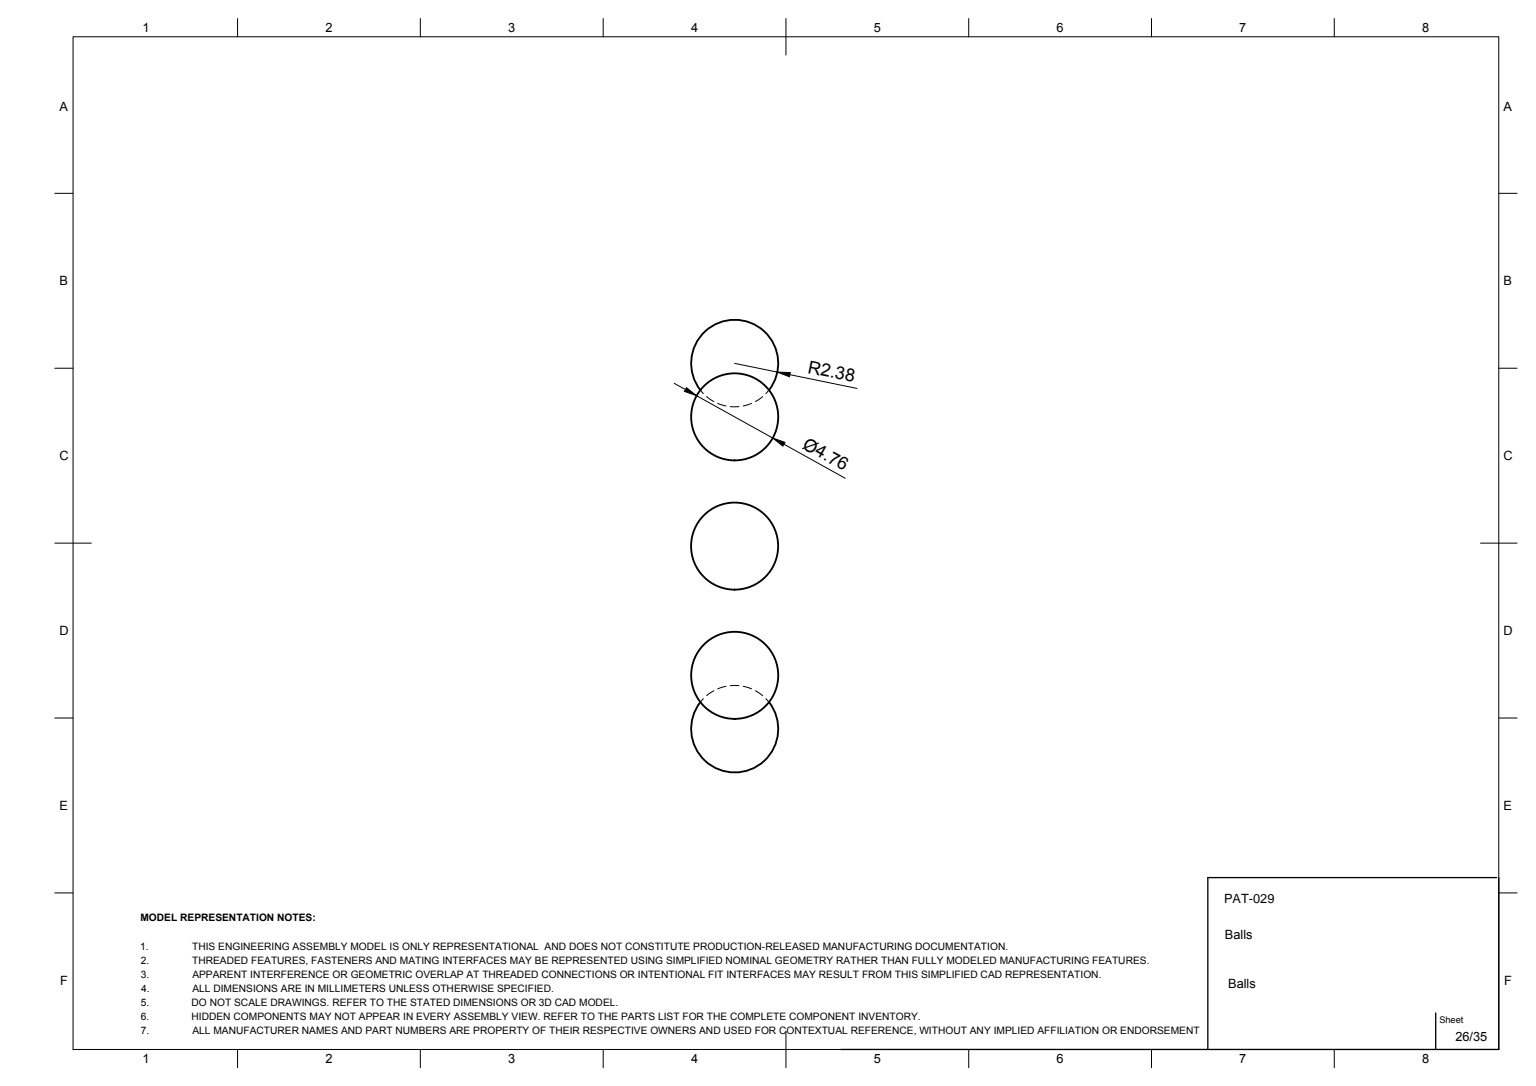
ISO-10303-21;
HEADER;
/* Generated by software containing ST-Developer
 * from STEP Tools, Inc. (www.steptools.com) 
 */

FILE_DESCRIPTION(
/* description */ ('Door-style hinge test fixture with detent'),
/* implementation_level */ '2;1');

FILE_NAME(
/* name */ 'Balls.step',
/* time_stamp */ '2026-10-28T03:24:57-07:00',
/* author */ (''),
/* organization */ (''),
/* preprocessor_version */ 'ST-DEVELOPER v20.2',
/* originating_system */ 'Autodesk Translation Framework v15.17.0.0',
/* authorisation */ '');

FILE_SCHEMA (('AUTOMOTIVE_DESIGN { 1 0 10303 214 3 1 1 }'));
ENDSEC;

DATA;
#10=MECHANICAL_DESIGN_GEOMETRIC_PRESENTATION_REPRESENTATION('',(#344,#345,#346,#347,#348,#349,#350,#351),#9813);
#243=SPHERICAL_SURFACE('',#5484,0.23815);
#244=SPHERICAL_SURFACE('',#5486,0.23815);
#245=SPHERICAL_SURFACE('',#5488,0.23815);
#246=SPHERICAL_SURFACE('',#5490,0.23815);
#247=SPHERICAL_SURFACE('',#5492,0.23815);
#248=SPHERICAL_SURFACE('',#5494,0.23815);
#249=SPHERICAL_SURFACE('',#5496,0.23815);
#250=SPHERICAL_SURFACE('',#5498,0.23815);
#281=SHAPE_REPRESENTATION_RELATIONSHIP('SRR','None',#9959,#312);
#312=ADVANCED_BREP_SHAPE_REPRESENTATION('',(#383,#384,#385,#386,#387,#388,
#389,#390),#9802);
#344=STYLED_ITEM('',(#10183),#383);
#345=STYLED_ITEM('',(#10183),#384);
#346=STYLED_ITEM('',(#10183),#385);
#347=STYLED_ITEM('',(#10183),#386);
#348=STYLED_ITEM('',(#10183),#387);
#349=STYLED_ITEM('',(#10183),#388);
#350=STYLED_ITEM('',(#10183),#389);
#351=STYLED_ITEM('',(#10183),#390);
#383=MANIFOLD_SOLID_BREP('Body1',#4776);
#384=MANIFOLD_SOLID_BREP('Body2',#4777);
#385=MANIFOLD_SOLID_BREP('Body3',#4778);
#386=MANIFOLD_SOLID_BREP('Body4',#4779);
#387=MANIFOLD_SOLID_BREP('Body5',#4780);
#388=MANIFOLD_SOLID_BREP('Body6',#4781);
#389=MANIFOLD_SOLID_BREP('Body7',#4782);
#390=MANIFOLD_SOLID_BREP('Body8',#4783);
#841=FACE_OUTER_BOUND('',#1199,.T.);
#842=FACE_OUTER_BOUND('',#1200,.T.);
#843=FACE_OUTER_BOUND('',#1201,.T.);
#844=FACE_OUTER_BOUND('',#1202,.T.);
#845=FACE_OUTER_BOUND('',#1203,.T.);
#846=FACE_OUTER_BOUND('',#1204,.T.);
#847=FACE_OUTER_BOUND('',#1205,.T.);
#848=FACE_OUTER_BOUND('',#1206,.T.);
#1199=EDGE_LOOP('',(#3963,#3964));
#1200=EDGE_LOOP('',(#3965,#3966));
#1201=EDGE_LOOP('',(#3967,#3968));
#1202=EDGE_LOOP('',(#3969,#3970));
#1203=EDGE_LOOP('',(#3971,#3972));
#1204=EDGE_LOOP('',(#3973,#3974));
#1205=EDGE_LOOP('',(#3975,#3976));
#1206=EDGE_LOOP('',(#3977,#3978));
#2118=CIRCLE('',#5485,0.23815);
#2119=CIRCLE('',#5487,0.23815);
#2120=CIRCLE('',#5489,0.23815);
#2121=CIRCLE('',#5491,0.23815);
#2122=CIRCLE('',#5493,0.23815);
#2123=CIRCLE('',#5495,0.23815);
#2124=CIRCLE('',#5497,0.23815);
#2125=CIRCLE('',#5499,0.23815);
#2472=VERTEX_POINT('',#8843);
#2473=VERTEX_POINT('',#8844);
#2474=VERTEX_POINT('',#8847);
#2475=VERTEX_POINT('',#8848);
#2476=VERTEX_POINT('',#8851);
#2477=VERTEX_POINT('',#8852);
#2478=VERTEX_POINT('',#8855);
#2479=VERTEX_POINT('',#8856);
#2480=VERTEX_POINT('',#8859);
#2481=VERTEX_POINT('',#8860);
#2482=VERTEX_POINT('',#8863);
#2483=VERTEX_POINT('',#8864);
#2484=VERTEX_POINT('',#8867);
#2485=VERTEX_POINT('',#8868);
#2486=VERTEX_POINT('',#8871);
#2487=VERTEX_POINT('',#8872);
#2998=EDGE_CURVE('',#2472,#2473,#2118,.T.);
#2999=EDGE_CURVE('',#2474,#2475,#2119,.T.);
#3000=EDGE_CURVE('',#2476,#2477,#2120,.T.);
#3001=EDGE_CURVE('',#2478,#2479,#2121,.T.);
#3002=EDGE_CURVE('',#2480,#2481,#2122,.T.);
#3003=EDGE_CURVE('',#2482,#2483,#2123,.T.);
#3004=EDGE_CURVE('',#2484,#2485,#2124,.T.);
#3005=EDGE_CURVE('',#2486,#2487,#2125,.T.);
#3963=ORIENTED_EDGE('',*,*,#2998,.T.);
#3964=ORIENTED_EDGE('',*,*,#2998,.F.);
#3965=ORIENTED_EDGE('',*,*,#2999,.T.);
#3966=ORIENTED_EDGE('',*,*,#2999,.F.);
#3967=ORIENTED_EDGE('',*,*,#3000,.T.);
#3968=ORIENTED_EDGE('',*,*,#3000,.F.);
#3969=ORIENTED_EDGE('',*,*,#3001,.T.);
#3970=ORIENTED_EDGE('',*,*,#3001,.F.);
#3971=ORIENTED_EDGE('',*,*,#3002,.T.);
#3972=ORIENTED_EDGE('',*,*,#3002,.F.);
#3973=ORIENTED_EDGE('',*,*,#3003,.T.);
#3974=ORIENTED_EDGE('',*,*,#3003,.F.);
#3975=ORIENTED_EDGE('',*,*,#3004,.T.);
#3976=ORIENTED_EDGE('',*,*,#3004,.F.);
#3977=ORIENTED_EDGE('',*,*,#3005,.T.);
#3978=ORIENTED_EDGE('',*,*,#3005,.F.);
#4646=ADVANCED_FACE('',(#841),#243,.T.);
#4647=ADVANCED_FACE('',(#842),#244,.T.);
#4648=ADVANCED_FACE('',(#843),#245,.T.);
#4649=ADVANCED_FACE('',(#844),#246,.T.);
#4650=ADVANCED_FACE('',(#845),#247,.T.);
#4651=ADVANCED_FACE('',(#846),#248,.T.);
#4652=ADVANCED_FACE('',(#847),#249,.T.);
#4653=ADVANCED_FACE('',(#848),#250,.T.);
#4776=CLOSED_SHELL('',(#4646));
#4777=CLOSED_SHELL('',(#4647));
#4778=CLOSED_SHELL('',(#4648));
#4779=CLOSED_SHELL('',(#4649));
#4780=CLOSED_SHELL('',(#4650));
#4781=CLOSED_SHELL('',(#4651));
#4782=CLOSED_SHELL('',(#4652));
#4783=CLOSED_SHELL('',(#4653));
#5483=AXIS2_PLACEMENT_3D('',#8841,#6674,#6675);
#5484=AXIS2_PLACEMENT_3D('',#8842,#6676,#6677);
#5485=AXIS2_PLACEMENT_3D('',#8845,#6678,#6679);
#5486=AXIS2_PLACEMENT_3D('',#8846,#6680,#6681);
#5487=AXIS2_PLACEMENT_3D('',#8849,#6682,#6683);
#5488=AXIS2_PLACEMENT_3D('',#8850,#6684,#6685);
#5489=AXIS2_PLACEMENT_3D('',#8853,#6686,#6687);
#5490=AXIS2_PLACEMENT_3D('',#8854,#6688,#6689);
#5491=AXIS2_PLACEMENT_3D('',#8857,#6690,#6691);
#5492=AXIS2_PLACEMENT_3D('',#8858,#6692,#6693);
#5493=AXIS2_PLACEMENT_3D('',#8861,#6694,#6695);
#5494=AXIS2_PLACEMENT_3D('',#8862,#6696,#6697);
#5495=AXIS2_PLACEMENT_3D('',#8865,#6698,#6699);
#5496=AXIS2_PLACEMENT_3D('',#8866,#6700,#6701);
#5497=AXIS2_PLACEMENT_3D('',#8869,#6702,#6703);
#5498=AXIS2_PLACEMENT_3D('',#8870,#6704,#6705);
#5499=AXIS2_PLACEMENT_3D('',#8873,#6706,#6707);
#6674=DIRECTION('axis',(0.,0.,1.));
#6675=DIRECTION('refdir',(1.,0.,0.));
#6676=DIRECTION('center_axis',(0.,0.,1.));
#6677=DIRECTION('ref_axis',(1.,0.,0.));
#6678=DIRECTION('center_axis',(1.22464679914735E-16,-1.,0.));
#6679=DIRECTION('ref_axis',(-1.,-1.22464679914735E-16,0.));
#6680=DIRECTION('center_axis',(0.707106781186548,0.,0.707106781186548));
#6681=DIRECTION('ref_axis',(0.707106781186548,0.,-0.707106781186548));
#6682=DIRECTION('center_axis',(8.65956056235494E-17,-1.,-8.65956056235493E-17));
#6683=DIRECTION('ref_axis',(-0.707106781186547,-1.22464679914735E-16,0.707106781186547));
#6684=DIRECTION('center_axis',(1.,0.,0.));
#6685=DIRECTION('ref_axis',(6.12323399573676E-17,0.,-1.));
#6686=DIRECTION('center_axis',(7.49879891330929E-33,-1.,-1.22464679914735E-16));
#6687=DIRECTION('ref_axis',(-6.12323399573676E-17,-1.22464679914735E-16,
1.));
#6688=DIRECTION('center_axis',(0.707106781186548,0.,-0.707106781186548));
#6689=DIRECTION('ref_axis',(-0.707106781186548,0.,-0.707106781186548));
#6690=DIRECTION('center_axis',(-8.65956056235493E-17,-1.,-8.65956056235494E-17));
#6691=DIRECTION('ref_axis',(0.707106781186547,-1.22464679914735E-16,0.707106781186547));
#6692=DIRECTION('center_axis',(0.,0.,-1.));
#6693=DIRECTION('ref_axis',(-1.,0.,-1.22464679914735E-16));
#6694=DIRECTION('center_axis',(-1.22464679914735E-16,-1.,-1.49975978266186E-32));
#6695=DIRECTION('ref_axis',(1.,-1.22464679914735E-16,1.22464679914735E-16));
#6696=DIRECTION('center_axis',(-0.707106781186547,0.,-0.707106781186548));
#6697=DIRECTION('ref_axis',(-0.707106781186548,0.,0.707106781186547));
#6698=DIRECTION('center_axis',(-8.65956056235493E-17,-1.,8.65956056235493E-17));
#6699=DIRECTION('ref_axis',(0.707106781186548,-1.22464679914735E-16,-0.707106781186547));
#6700=DIRECTION('center_axis',(-1.,0.,0.));
#6701=DIRECTION('ref_axis',(-1.83697019872103E-16,0.,1.));
#6702=DIRECTION('center_axis',(-2.24963967399279E-32,-1.,1.22464679914735E-16));
#6703=DIRECTION('ref_axis',(1.83697019872103E-16,-1.22464679914735E-16,
-1.));
#6704=DIRECTION('center_axis',(-0.707106781186548,0.,0.707106781186548));
#6705=DIRECTION('ref_axis',(0.707106781186547,0.,0.707106781186548));
#6706=DIRECTION('center_axis',(8.65956056235493E-17,-1.,8.65956056235493E-17));
#6707=DIRECTION('ref_axis',(-0.707106781186547,-1.22464679914735E-16,-0.707106781186548));
#8841=CARTESIAN_POINT('',(0.,0.,0.));
#8842=CARTESIAN_POINT('Origin',(1.,0.,0.));
#8843=CARTESIAN_POINT('',(1.,-1.78583896120461E-33,0.23815));
#8844=CARTESIAN_POINT('',(1.,-1.78583896120461E-33,-0.23815));
#8845=CARTESIAN_POINT('Origin',(1.,0.,0.));
#8846=CARTESIAN_POINT('Origin',(0.707106781186548,0.,-0.707106781186547));
#8847=CARTESIAN_POINT('',(0.875504261126124,-1.78583896120461E-33,-0.538709301246971));
#8848=CARTESIAN_POINT('',(0.538709301246971,-1.78583896120461E-33,-0.875504261126124));
#8849=CARTESIAN_POINT('Origin',(0.707106781186548,0.,-0.707106781186547));
#8850=CARTESIAN_POINT('Origin',(6.12323399573677E-17,0.,-1.));
#8851=CARTESIAN_POINT('',(0.23815,-1.78583896120461E-33,-1.));
#8852=CARTESIAN_POINT('',(-0.23815,-1.78583896120461E-33,-1.));
#8853=CARTESIAN_POINT('Origin',(6.12323399573677E-17,0.,-1.));
#8854=CARTESIAN_POINT('Origin',(-0.707106781186547,0.,-0.707106781186548));
#8855=CARTESIAN_POINT('',(-0.538709301246971,-1.78583896120461E-33,-0.875504261126124));
#8856=CARTESIAN_POINT('',(-0.875504261126124,-1.78583896120461E-33,-0.538709301246971));
#8857=CARTESIAN_POINT('Origin',(-0.707106781186547,0.,-0.707106781186548));
#8858=CARTESIAN_POINT('Origin',(-1.,0.,-1.22464679914735E-16));
#8859=CARTESIAN_POINT('',(-1.,-1.78583896120461E-33,-0.23815));
#8860=CARTESIAN_POINT('',(-1.,-1.78583896120461E-33,0.23815));
#8861=CARTESIAN_POINT('Origin',(-1.,0.,-1.22464679914735E-16));
#8862=CARTESIAN_POINT('Origin',(-0.707106781186548,0.,0.707106781186547));
#8863=CARTESIAN_POINT('',(-0.875504261126124,-7.94881478324376E-33,0.538709301246971));
#8864=CARTESIAN_POINT('',(-0.538709301246971,4.37713686083455E-33,0.875504261126124));
#8865=CARTESIAN_POINT('Origin',(-0.707106781186548,0.,0.707106781186547));
#8866=CARTESIAN_POINT('Origin',(-1.83697019872103E-16,0.,1.));
#8867=CARTESIAN_POINT('',(-0.23815,-1.78583896120461E-33,1.));
#8868=CARTESIAN_POINT('',(0.23815,-1.78583896120461E-33,1.));
#8869=CARTESIAN_POINT('Origin',(-1.83697019872103E-16,0.,1.));
#8870=CARTESIAN_POINT('Origin',(0.707106781186547,0.,0.707106781186548));
#8871=CARTESIAN_POINT('',(0.538709301246971,-4.86732687222419E-33,0.875504261126124));
#8872=CARTESIAN_POINT('',(0.875504261126124,1.29564894981497E-33,0.538709301246971));
#8873=CARTESIAN_POINT('Origin',(0.707106781186547,0.,0.707106781186548));
#9766=UNCERTAINTY_MEASURE_WITH_UNIT(LENGTH_MEASURE(0.001),#9814,
'DISTANCE_ACCURACY_VALUE',
'Maximum model space distance between geometric entities at asserted c
onnectivities');
#9777=UNCERTAINTY_MEASURE_WITH_UNIT(LENGTH_MEASURE(0.001),#9814,
'DISTANCE_ACCURACY_VALUE',
'Maximum model space distance between geometric entities at asserted c
onnectivities');
#9802=(
GEOMETRIC_REPRESENTATION_CONTEXT(3)
GLOBAL_UNCERTAINTY_ASSIGNED_CONTEXT((#9766))
GLOBAL_UNIT_ASSIGNED_CONTEXT((#9814,#9816,#9817))
REPRESENTATION_CONTEXT('','3D')
);
#9813=(
GEOMETRIC_REPRESENTATION_CONTEXT(3)
GLOBAL_UNCERTAINTY_ASSIGNED_CONTEXT((#9777))
GLOBAL_UNIT_ASSIGNED_CONTEXT((#9814,#9816,#9817))
REPRESENTATION_CONTEXT('','3D')
);
#9814=(
LENGTH_UNIT()
NAMED_UNIT(*)
SI_UNIT(.CENTI.,.METRE.)
);
#9816=(
NAMED_UNIT(*)
PLANE_ANGLE_UNIT()
SI_UNIT($,.RADIAN.)
);
#9817=(
NAMED_UNIT(*)
SI_UNIT($,.STERADIAN.)
SOLID_ANGLE_UNIT()
);
#9842=SHAPE_DEFINITION_REPRESENTATION(#9877,#9959);
#9877=PRODUCT_DEFINITION_SHAPE('',$,#9995);
#9959=SHAPE_REPRESENTATION('',(#5483),#9802);
#9970=PRODUCT_DEFINITION_CONTEXT('part definition',#10077,'design');
#9995=PRODUCT_DEFINITION('Balls','Balls',#10030,#9970);
#10030=PRODUCT_DEFINITION_FORMATION('',$,#10103);
#10077=APPLICATION_CONTEXT(
'Core Data for Automotive Mechanical Design Process');
#10078=PRODUCT_CONTEXT('part definition',#10077,'mechanical');
#10103=PRODUCT('Balls','Balls','Balls',(#10078));
#10177=COLOUR_RGB('Grey',0.48,0.52,0.57);
#10178=FILL_AREA_STYLE_COLOUR('',#10177);
#10179=FILL_AREA_STYLE('',(#10178));
#10180=SURFACE_STYLE_FILL_AREA(#10179);
#10181=SURFACE_SIDE_STYLE('',(#10180));
#10182=SURFACE_STYLE_USAGE(.BOTH.,#10181);
#10183=PRESENTATION_STYLE_ASSIGNMENT((#10182));
ENDSEC;
END-ISO-10303-21;
